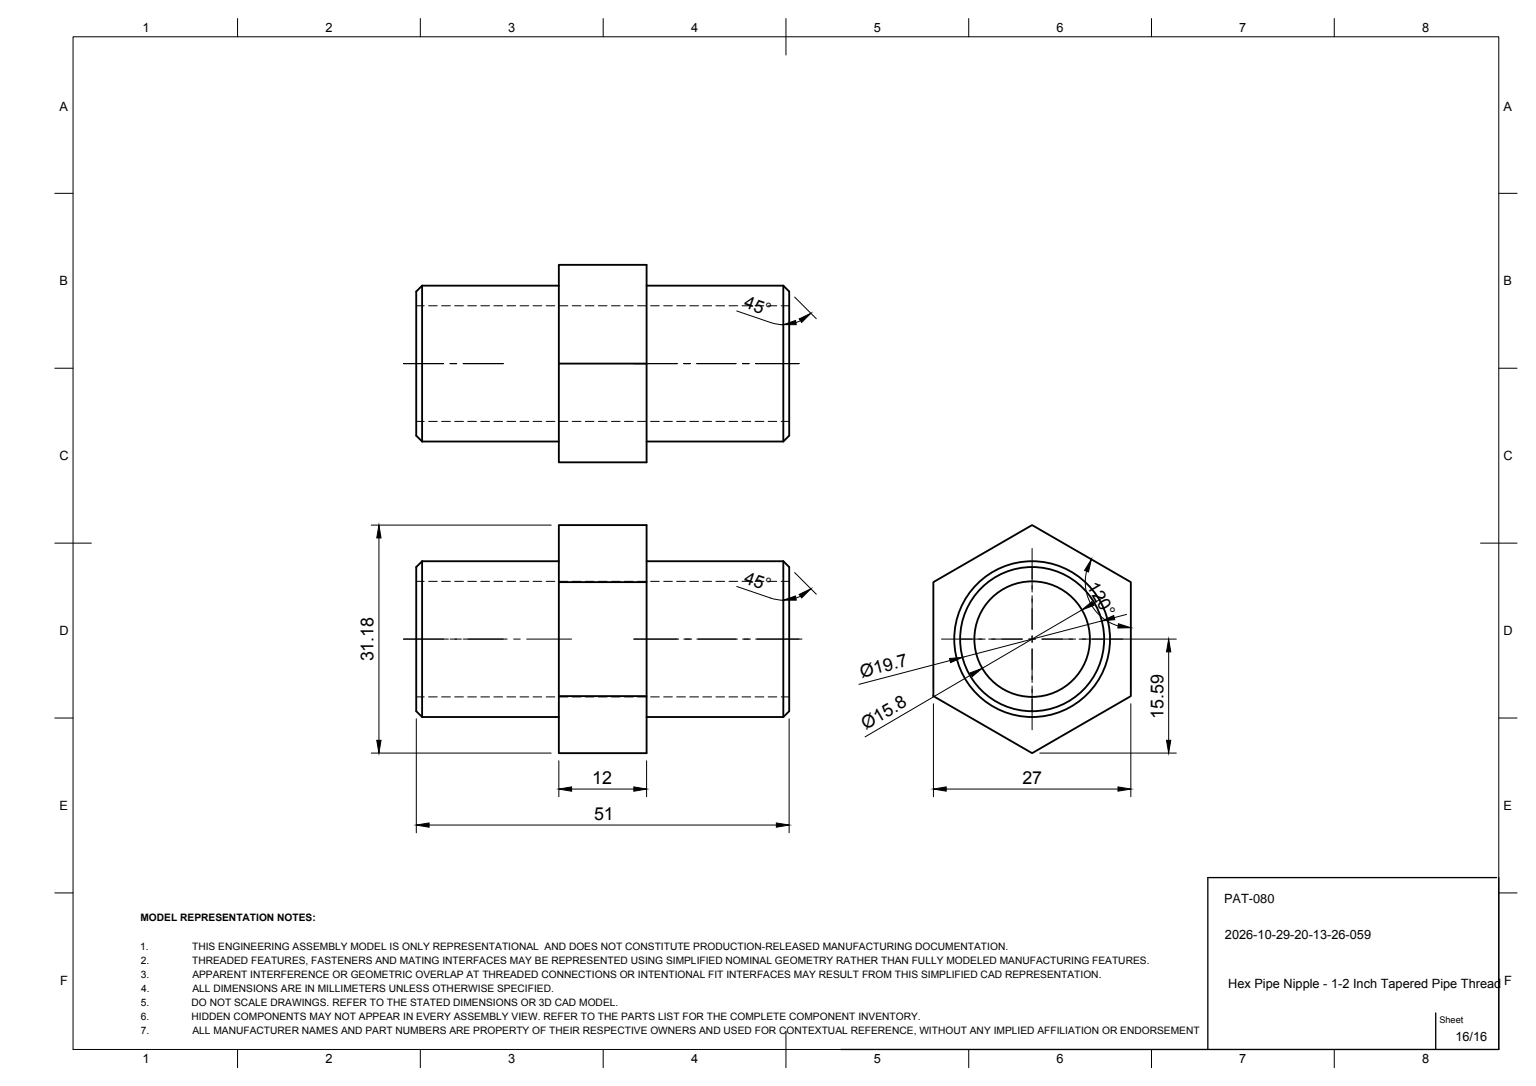
ISO-10303-21;
HEADER;
/* Generated by software containing ST-Developer
 * from STEP Tools, Inc. (www.steptools.com) 
 */

FILE_DESCRIPTION(
/* description */ ('PAT-080'),
/* implementation_level */ '2;1');

FILE_NAME(
/* name */ 'Hex Pipe Nipple - 1-2 Inch Tapered Pipe Thread.step',
/* time_stamp */ '2026-10-29T20:13:47-07:00',
/* author */ (''),
/* organization */ (''),
/* preprocessor_version */ 'ST-DEVELOPER v20.2',
/* originating_system */ 'Autodesk Translation Framework v15.17.0.0',
/* authorisation */ '');

FILE_SCHEMA (('AUTOMOTIVE_DESIGN { 1 0 10303 214 3 1 1 }'));
ENDSEC;

DATA;
#10=MECHANICAL_DESIGN_GEOMETRIC_PRESENTATION_REPRESENTATION('',(#261),#6878);
#194=CONICAL_SURFACE('',#4435,1.025,0.785398163397448);
#195=CONICAL_SURFACE('',#4438,1.025,0.785398163397448);
#223=SHAPE_REPRESENTATION_RELATIONSHIP('SRR','None',#6979,#242);
#242=ADVANCED_BREP_SHAPE_REPRESENTATION('',(#278),#6874);
#261=STYLED_ITEM('',(#7115),#278);
#278=MANIFOLD_SOLID_BREP('Body1',#3879);
#348=FACE_BOUND('',#973,.T.);
#349=FACE_BOUND('',#975,.T.);
#350=FACE_BOUND('',#984,.T.);
#351=FACE_BOUND('',#989,.T.);
#469=PLANE('',#4420);
#470=PLANE('',#4422);
#471=PLANE('',#4424);
#472=PLANE('',#4425);
#473=PLANE('',#4426);
#474=PLANE('',#4427);
#475=PLANE('',#4428);
#476=PLANE('',#4429);
#477=PLANE('',#4432);
#478=PLANE('',#4440);
#679=FACE_OUTER_BOUND('',#972,.T.);
#680=FACE_OUTER_BOUND('',#974,.T.);
#681=FACE_OUTER_BOUND('',#976,.T.);
#682=FACE_OUTER_BOUND('',#977,.T.);
#683=FACE_OUTER_BOUND('',#978,.T.);
#684=FACE_OUTER_BOUND('',#979,.T.);
#685=FACE_OUTER_BOUND('',#980,.T.);
#686=FACE_OUTER_BOUND('',#981,.T.);
#687=FACE_OUTER_BOUND('',#982,.T.);
#688=FACE_OUTER_BOUND('',#983,.T.);
#689=FACE_OUTER_BOUND('',#985,.T.);
#690=FACE_OUTER_BOUND('',#986,.T.);
#691=FACE_OUTER_BOUND('',#987,.T.);
#692=FACE_OUTER_BOUND('',#988,.T.);
#693=FACE_OUTER_BOUND('',#990,.T.);
#972=EDGE_LOOP('',(#3382,#3383,#3384,#3385,#3386,#3387));
#973=EDGE_LOOP('',(#3388));
#974=EDGE_LOOP('',(#3389,#3390,#3391,#3392,#3393,#3394));
#975=EDGE_LOOP('',(#3395));
#976=EDGE_LOOP('',(#3396,#3397,#3398,#3399));
#977=EDGE_LOOP('',(#3400,#3401,#3402,#3403));
#978=EDGE_LOOP('',(#3404,#3405,#3406,#3407));
#979=EDGE_LOOP('',(#3408,#3409,#3410,#3411));
#980=EDGE_LOOP('',(#3412,#3413,#3414,#3415));
#981=EDGE_LOOP('',(#3416,#3417,#3418,#3419));
#982=EDGE_LOOP('',(#3420,#3421,#3422,#3423));
#983=EDGE_LOOP('',(#3424));
#984=EDGE_LOOP('',(#3425));
#985=EDGE_LOOP('',(#3426,#3427,#3428,#3429));
#986=EDGE_LOOP('',(#3430,#3431,#3432,#3433));
#987=EDGE_LOOP('',(#3434,#3435,#3436,#3437));
#988=EDGE_LOOP('',(#3438));
#989=EDGE_LOOP('',(#3439));
#990=EDGE_LOOP('',(#3440,#3441,#3442,#3443));
#1285=LINE('',#6572,#1600);
#1286=LINE('',#6574,#1601);
#1287=LINE('',#6576,#1602);
#1288=LINE('',#6578,#1603);
#1289=LINE('',#6580,#1604);
#1290=LINE('',#6581,#1605);
#1291=LINE('',#6587,#1606);
#1292=LINE('',#6589,#1607);
#1293=LINE('',#6591,#1608);
#1294=LINE('',#6593,#1609);
#1295=LINE('',#6595,#1610);
#1296=LINE('',#6596,#1611);
#1297=LINE('',#6600,#1612);
#1298=LINE('',#6601,#1613);
#1299=LINE('',#6603,#1614);
#1300=LINE('',#6605,#1615);
#1301=LINE('',#6607,#1616);
#1302=LINE('',#6609,#1617);
#1303=LINE('',#6613,#1618);
#1304=LINE('',#6621,#1619);
#1305=LINE('',#6625,#1620);
#1306=LINE('',#6629,#1621);
#1307=LINE('',#6634,#1622);
#1600=VECTOR('',#5445,1.);
#1601=VECTOR('',#5446,1.);
#1602=VECTOR('',#5447,1.);
#1603=VECTOR('',#5448,1.);
#1604=VECTOR('',#5449,1.);
#1605=VECTOR('',#5450,1.);
#1606=VECTOR('',#5455,1.);
#1607=VECTOR('',#5456,1.);
#1608=VECTOR('',#5457,1.);
#1609=VECTOR('',#5458,1.);
#1610=VECTOR('',#5459,1.);
#1611=VECTOR('',#5460,1.);
#1612=VECTOR('',#5465,1.);
#1613=VECTOR('',#5466,1.);
#1614=VECTOR('',#5469,1.);
#1615=VECTOR('',#5472,1.);
#1616=VECTOR('',#5475,1.);
#1617=VECTOR('',#5478,1.);
#1618=VECTOR('',#5483,1.065);
#1619=VECTOR('',#5494,1.025);
#1620=VECTOR('',#5499,1.065);
#1621=VECTOR('',#5504,1.025);
#1622=VECTOR('',#5511,0.79);
#1786=CIRCLE('',#4421,1.065);
#1787=CIRCLE('',#4423,1.065);
#1788=CIRCLE('',#4431,1.065);
#1789=CIRCLE('',#4433,0.985);
#1790=CIRCLE('',#4434,0.79);
#1791=CIRCLE('',#4437,1.065);
#1792=CIRCLE('',#4439,0.985);
#1793=CIRCLE('',#4441,0.79);
#2067=VERTEX_POINT('',#6570);
#2068=VERTEX_POINT('',#6571);
#2069=VERTEX_POINT('',#6573);
#2070=VERTEX_POINT('',#6575);
#2071=VERTEX_POINT('',#6577);
#2072=VERTEX_POINT('',#6579);
#2073=VERTEX_POINT('',#6582);
#2074=VERTEX_POINT('',#6585);
#2075=VERTEX_POINT('',#6586);
#2076=VERTEX_POINT('',#6588);
#2077=VERTEX_POINT('',#6590);
#2078=VERTEX_POINT('',#6592);
#2079=VERTEX_POINT('',#6594);
#2080=VERTEX_POINT('',#6597);
#2081=VERTEX_POINT('',#6612);
#2082=VERTEX_POINT('',#6616);
#2083=VERTEX_POINT('',#6618);
#2084=VERTEX_POINT('',#6623);
#2085=VERTEX_POINT('',#6627);
#2086=VERTEX_POINT('',#6631);
#2514=EDGE_CURVE('',#2067,#2068,#1285,.T.);
#2515=EDGE_CURVE('',#2068,#2069,#1286,.T.);
#2516=EDGE_CURVE('',#2069,#2070,#1287,.T.);
#2517=EDGE_CURVE('',#2070,#2071,#1288,.T.);
#2518=EDGE_CURVE('',#2071,#2072,#1289,.T.);
#2519=EDGE_CURVE('',#2072,#2067,#1290,.T.);
#2520=EDGE_CURVE('',#2073,#2073,#1786,.T.);
#2521=EDGE_CURVE('',#2074,#2075,#1291,.T.);
#2522=EDGE_CURVE('',#2075,#2076,#1292,.T.);
#2523=EDGE_CURVE('',#2076,#2077,#1293,.T.);
#2524=EDGE_CURVE('',#2077,#2078,#1294,.T.);
#2525=EDGE_CURVE('',#2078,#2079,#1295,.T.);
#2526=EDGE_CURVE('',#2079,#2074,#1296,.T.);
#2527=EDGE_CURVE('',#2080,#2080,#1787,.T.);
#2528=EDGE_CURVE('',#2074,#2068,#1297,.T.);
#2529=EDGE_CURVE('',#2069,#2079,#1298,.T.);
#2530=EDGE_CURVE('',#2070,#2078,#1299,.T.);
#2531=EDGE_CURVE('',#2071,#2077,#1300,.T.);
#2532=EDGE_CURVE('',#2072,#2076,#1301,.T.);
#2533=EDGE_CURVE('',#2067,#2075,#1302,.T.);
#2534=EDGE_CURVE('',#2080,#2081,#1303,.T.);
#2535=EDGE_CURVE('',#2081,#2081,#1788,.T.);
#2536=EDGE_CURVE('',#2082,#2082,#1789,.T.);
#2537=EDGE_CURVE('',#2083,#2083,#1790,.T.);
#2538=EDGE_CURVE('',#2081,#2082,#1304,.T.);
#2539=EDGE_CURVE('',#2084,#2084,#1791,.T.);
#2540=EDGE_CURVE('',#2084,#2073,#1305,.T.);
#2541=EDGE_CURVE('',#2085,#2085,#1792,.T.);
#2542=EDGE_CURVE('',#2085,#2084,#1306,.T.);
#2543=EDGE_CURVE('',#2086,#2086,#1793,.T.);
#2544=EDGE_CURVE('',#2086,#2083,#1307,.T.);
#3382=ORIENTED_EDGE('',*,*,#2514,.T.);
#3383=ORIENTED_EDGE('',*,*,#2515,.T.);
#3384=ORIENTED_EDGE('',*,*,#2516,.T.);
#3385=ORIENTED_EDGE('',*,*,#2517,.T.);
#3386=ORIENTED_EDGE('',*,*,#2518,.T.);
#3387=ORIENTED_EDGE('',*,*,#2519,.T.);
#3388=ORIENTED_EDGE('',*,*,#2520,.F.);
#3389=ORIENTED_EDGE('',*,*,#2521,.T.);
#3390=ORIENTED_EDGE('',*,*,#2522,.T.);
#3391=ORIENTED_EDGE('',*,*,#2523,.T.);
#3392=ORIENTED_EDGE('',*,*,#2524,.T.);
#3393=ORIENTED_EDGE('',*,*,#2525,.T.);
#3394=ORIENTED_EDGE('',*,*,#2526,.T.);
#3395=ORIENTED_EDGE('',*,*,#2527,.F.);
#3396=ORIENTED_EDGE('',*,*,#2528,.F.);
#3397=ORIENTED_EDGE('',*,*,#2526,.F.);
#3398=ORIENTED_EDGE('',*,*,#2529,.F.);
#3399=ORIENTED_EDGE('',*,*,#2515,.F.);
#3400=ORIENTED_EDGE('',*,*,#2529,.T.);
#3401=ORIENTED_EDGE('',*,*,#2525,.F.);
#3402=ORIENTED_EDGE('',*,*,#2530,.F.);
#3403=ORIENTED_EDGE('',*,*,#2516,.F.);
#3404=ORIENTED_EDGE('',*,*,#2530,.T.);
#3405=ORIENTED_EDGE('',*,*,#2524,.F.);
#3406=ORIENTED_EDGE('',*,*,#2531,.F.);
#3407=ORIENTED_EDGE('',*,*,#2517,.F.);
#3408=ORIENTED_EDGE('',*,*,#2531,.T.);
#3409=ORIENTED_EDGE('',*,*,#2523,.F.);
#3410=ORIENTED_EDGE('',*,*,#2532,.F.);
#3411=ORIENTED_EDGE('',*,*,#2518,.F.);
#3412=ORIENTED_EDGE('',*,*,#2532,.T.);
#3413=ORIENTED_EDGE('',*,*,#2522,.F.);
#3414=ORIENTED_EDGE('',*,*,#2533,.F.);
#3415=ORIENTED_EDGE('',*,*,#2519,.F.);
#3416=ORIENTED_EDGE('',*,*,#2533,.T.);
#3417=ORIENTED_EDGE('',*,*,#2521,.F.);
#3418=ORIENTED_EDGE('',*,*,#2528,.T.);
#3419=ORIENTED_EDGE('',*,*,#2514,.F.);
#3420=ORIENTED_EDGE('',*,*,#2527,.T.);
#3421=ORIENTED_EDGE('',*,*,#2534,.T.);
#3422=ORIENTED_EDGE('',*,*,#2535,.T.);
#3423=ORIENTED_EDGE('',*,*,#2534,.F.);
#3424=ORIENTED_EDGE('',*,*,#2536,.F.);
#3425=ORIENTED_EDGE('',*,*,#2537,.T.);
#3426=ORIENTED_EDGE('',*,*,#2535,.F.);
#3427=ORIENTED_EDGE('',*,*,#2538,.T.);
#3428=ORIENTED_EDGE('',*,*,#2536,.T.);
#3429=ORIENTED_EDGE('',*,*,#2538,.F.);
#3430=ORIENTED_EDGE('',*,*,#2539,.F.);
#3431=ORIENTED_EDGE('',*,*,#2540,.T.);
#3432=ORIENTED_EDGE('',*,*,#2520,.T.);
#3433=ORIENTED_EDGE('',*,*,#2540,.F.);
#3434=ORIENTED_EDGE('',*,*,#2541,.F.);
#3435=ORIENTED_EDGE('',*,*,#2542,.T.);
#3436=ORIENTED_EDGE('',*,*,#2539,.T.);
#3437=ORIENTED_EDGE('',*,*,#2542,.F.);
#3438=ORIENTED_EDGE('',*,*,#2541,.T.);
#3439=ORIENTED_EDGE('',*,*,#2543,.F.);
#3440=ORIENTED_EDGE('',*,*,#2543,.T.);
#3441=ORIENTED_EDGE('',*,*,#2544,.T.);
#3442=ORIENTED_EDGE('',*,*,#2537,.F.);
#3443=ORIENTED_EDGE('',*,*,#2544,.F.);
#3628=CYLINDRICAL_SURFACE('',#4430,1.065);
#3629=CYLINDRICAL_SURFACE('',#4436,1.065);
#3630=CYLINDRICAL_SURFACE('',#4442,0.79);
#3815=ADVANCED_FACE('',(#679,#348),#469,.F.);
#3816=ADVANCED_FACE('',(#680,#349),#470,.T.);
#3817=ADVANCED_FACE('',(#681),#471,.T.);
#3818=ADVANCED_FACE('',(#682),#472,.T.);
#3819=ADVANCED_FACE('',(#683),#473,.T.);
#3820=ADVANCED_FACE('',(#684),#474,.T.);
#3821=ADVANCED_FACE('',(#685),#475,.T.);
#3822=ADVANCED_FACE('',(#686),#476,.T.);
#3823=ADVANCED_FACE('',(#687),#3628,.T.);
#3824=ADVANCED_FACE('',(#688,#350),#477,.T.);
#3825=ADVANCED_FACE('',(#689),#194,.T.);
#3826=ADVANCED_FACE('',(#690),#3629,.T.);
#3827=ADVANCED_FACE('',(#691),#195,.T.);
#3828=ADVANCED_FACE('',(#692,#351),#478,.T.);
#3829=ADVANCED_FACE('',(#693),#3630,.F.);
#3879=CLOSED_SHELL('',(#3815,#3816,#3817,#3818,#3819,#3820,#3821,#3822,
#3823,#3824,#3825,#3826,#3827,#3828,#3829));
#4419=AXIS2_PLACEMENT_3D('',#6568,#5441,#5442);
#4420=AXIS2_PLACEMENT_3D('',#6569,#5443,#5444);
#4421=AXIS2_PLACEMENT_3D('',#6583,#5451,#5452);
#4422=AXIS2_PLACEMENT_3D('',#6584,#5453,#5454);
#4423=AXIS2_PLACEMENT_3D('',#6598,#5461,#5462);
#4424=AXIS2_PLACEMENT_3D('',#6599,#5463,#5464);
#4425=AXIS2_PLACEMENT_3D('',#6602,#5467,#5468);
#4426=AXIS2_PLACEMENT_3D('',#6604,#5470,#5471);
#4427=AXIS2_PLACEMENT_3D('',#6606,#5473,#5474);
#4428=AXIS2_PLACEMENT_3D('',#6608,#5476,#5477);
#4429=AXIS2_PLACEMENT_3D('',#6610,#5479,#5480);
#4430=AXIS2_PLACEMENT_3D('',#6611,#5481,#5482);
#4431=AXIS2_PLACEMENT_3D('',#6614,#5484,#5485);
#4432=AXIS2_PLACEMENT_3D('',#6615,#5486,#5487);
#4433=AXIS2_PLACEMENT_3D('',#6617,#5488,#5489);
#4434=AXIS2_PLACEMENT_3D('',#6619,#5490,#5491);
#4435=AXIS2_PLACEMENT_3D('',#6620,#5492,#5493);
#4436=AXIS2_PLACEMENT_3D('',#6622,#5495,#5496);
#4437=AXIS2_PLACEMENT_3D('',#6624,#5497,#5498);
#4438=AXIS2_PLACEMENT_3D('',#6626,#5500,#5501);
#4439=AXIS2_PLACEMENT_3D('',#6628,#5502,#5503);
#4440=AXIS2_PLACEMENT_3D('',#6630,#5505,#5506);
#4441=AXIS2_PLACEMENT_3D('',#6632,#5507,#5508);
#4442=AXIS2_PLACEMENT_3D('',#6633,#5509,#5510);
#5441=DIRECTION('axis',(0.,0.,1.));
#5442=DIRECTION('refdir',(1.,0.,0.));
#5443=DIRECTION('center_axis',(0.,1.,0.));
#5444=DIRECTION('ref_axis',(1.,0.,0.));
#5445=DIRECTION('',(-0.5,0.,0.866025403784439));
#5446=DIRECTION('',(-1.,0.,-2.84883360945713E-16));
#5447=DIRECTION('',(-0.5,0.,-0.866025403784439));
#5448=DIRECTION('',(0.5,0.,-0.866025403784439));
#5449=DIRECTION('',(1.,0.,0.));
#5450=DIRECTION('',(0.5,0.,0.866025403784439));
#5451=DIRECTION('center_axis',(0.,-1.,0.));
#5452=DIRECTION('ref_axis',(1.,0.,0.));
#5453=DIRECTION('center_axis',(0.,1.,0.));
#5454=DIRECTION('ref_axis',(1.,0.,0.));
#5455=DIRECTION('',(0.5,0.,-0.866025403784439));
#5456=DIRECTION('',(-0.5,0.,-0.866025403784439));
#5457=DIRECTION('',(-1.,0.,0.));
#5458=DIRECTION('',(-0.5,0.,0.866025403784439));
#5459=DIRECTION('',(0.5,0.,0.866025403784439));
#5460=DIRECTION('',(1.,0.,2.84883360945713E-16));
#5461=DIRECTION('center_axis',(0.,1.,0.));
#5462=DIRECTION('ref_axis',(1.,0.,0.));
#5463=DIRECTION('center_axis',(-2.84883360945713E-16,0.,1.));
#5464=DIRECTION('ref_axis',(1.,0.,2.84883360945713E-16));
#5465=DIRECTION('',(0.,-1.,0.));
#5466=DIRECTION('',(0.,1.,0.));
#5467=DIRECTION('center_axis',(-0.866025403784439,0.,0.5));
#5468=DIRECTION('ref_axis',(0.5,0.,0.866025403784439));
#5469=DIRECTION('',(0.,1.,0.));
#5470=DIRECTION('center_axis',(-0.866025403784439,0.,-0.5));
#5471=DIRECTION('ref_axis',(-0.5,0.,0.866025403784439));
#5472=DIRECTION('',(0.,1.,0.));
#5473=DIRECTION('center_axis',(0.,0.,-1.));
#5474=DIRECTION('ref_axis',(-1.,0.,0.));
#5475=DIRECTION('',(0.,1.,0.));
#5476=DIRECTION('center_axis',(0.866025403784439,0.,-0.5));
#5477=DIRECTION('ref_axis',(-0.5,0.,-0.866025403784439));
#5478=DIRECTION('',(0.,1.,0.));
#5479=DIRECTION('center_axis',(0.866025403784439,0.,0.5));
#5480=DIRECTION('ref_axis',(0.5,0.,-0.866025403784439));
#5481=DIRECTION('center_axis',(0.,-1.,0.));
#5482=DIRECTION('ref_axis',(1.,0.,0.));
#5483=DIRECTION('',(0.,1.,0.));
#5484=DIRECTION('center_axis',(0.,-1.,0.));
#5485=DIRECTION('ref_axis',(1.,0.,0.));
#5486=DIRECTION('center_axis',(0.,1.,0.));
#5487=DIRECTION('ref_axis',(0.,0.,1.));
#5488=DIRECTION('center_axis',(0.,-1.,0.));
#5489=DIRECTION('ref_axis',(1.,0.,0.));
#5490=DIRECTION('center_axis',(0.,-1.,0.));
#5491=DIRECTION('ref_axis',(1.,0.,0.));
#5492=DIRECTION('center_axis',(0.,-1.,0.));
#5493=DIRECTION('ref_axis',(1.,0.,0.));
#5494=DIRECTION('',(0.707106781186547,0.707106781186548,8.65956056235493E-17));
#5495=DIRECTION('center_axis',(0.,-1.,0.));
#5496=DIRECTION('ref_axis',(1.,0.,0.));
#5497=DIRECTION('center_axis',(0.,-1.,0.));
#5498=DIRECTION('ref_axis',(1.,0.,0.));
#5499=DIRECTION('',(0.,1.,0.));
#5500=DIRECTION('center_axis',(0.,1.,0.));
#5501=DIRECTION('ref_axis',(1.,0.,0.));
#5502=DIRECTION('center_axis',(0.,-1.,0.));
#5503=DIRECTION('ref_axis',(1.,0.,0.));
#5504=DIRECTION('',(-0.707106781186547,0.707106781186548,-8.65956056235493E-17));
#5505=DIRECTION('center_axis',(0.,-1.,0.));
#5506=DIRECTION('ref_axis',(0.,0.,-1.));
#5507=DIRECTION('center_axis',(0.,-1.,0.));
#5508=DIRECTION('ref_axis',(1.,0.,0.));
#5509=DIRECTION('center_axis',(0.,-1.,0.));
#5510=DIRECTION('ref_axis',(1.,0.,0.));
#5511=DIRECTION('',(0.,1.,0.));
#6568=CARTESIAN_POINT('',(0.,0.,0.));
#6569=CARTESIAN_POINT('Origin',(0.,-0.6,0.));
#6570=CARTESIAN_POINT('',(1.55884572681199,-0.6,0.));
#6571=CARTESIAN_POINT('',(0.779422863405995,-0.6,1.35));
#6572=CARTESIAN_POINT('',(0.779422863405995,-0.6,1.35));
#6573=CARTESIAN_POINT('',(-0.779422863405996,-0.6,1.35));
#6574=CARTESIAN_POINT('',(-0.779422863405996,-0.6,1.35));
#6575=CARTESIAN_POINT('',(-1.55884572681199,-0.6,-1.90903542970483E-16));
#6576=CARTESIAN_POINT('',(-1.55884572681199,-0.6,-1.90903542970483E-16));
#6577=CARTESIAN_POINT('',(-0.779422863405995,-0.6,-1.35));
#6578=CARTESIAN_POINT('',(-0.779422863405995,-0.6,-1.35));
#6579=CARTESIAN_POINT('',(0.779422863405995,-0.6,-1.35));
#6580=CARTESIAN_POINT('',(0.779422863405995,-0.6,-1.35));
#6581=CARTESIAN_POINT('',(1.55884572681199,-0.6,0.));
#6582=CARTESIAN_POINT('',(-1.065,-0.6,-1.30424884109193E-16));
#6583=CARTESIAN_POINT('Origin',(0.,-0.6,0.));
#6584=CARTESIAN_POINT('Origin',(0.,0.6,0.));
#6585=CARTESIAN_POINT('',(0.779422863405995,0.6,1.35));
#6586=CARTESIAN_POINT('',(1.55884572681199,0.6,0.));
#6587=CARTESIAN_POINT('',(0.779422863405995,0.6,1.35));
#6588=CARTESIAN_POINT('',(0.779422863405995,0.6,-1.35));
#6589=CARTESIAN_POINT('',(1.55884572681199,0.6,0.));
#6590=CARTESIAN_POINT('',(-0.779422863405995,0.6,-1.35));
#6591=CARTESIAN_POINT('',(0.779422863405995,0.6,-1.35));
#6592=CARTESIAN_POINT('',(-1.55884572681199,0.6,-1.90903542970483E-16));
#6593=CARTESIAN_POINT('',(-0.779422863405995,0.6,-1.35));
#6594=CARTESIAN_POINT('',(-0.779422863405996,0.6,1.35));
#6595=CARTESIAN_POINT('',(-1.55884572681199,0.6,-1.90903542970483E-16));
#6596=CARTESIAN_POINT('',(-0.779422863405996,0.6,1.35));
#6597=CARTESIAN_POINT('',(-1.065,0.6,1.30424884109193E-16));
#6598=CARTESIAN_POINT('Origin',(0.,0.6,0.));
#6599=CARTESIAN_POINT('Origin',(-0.779422863405996,0.,1.35));
#6600=CARTESIAN_POINT('',(0.779422863405995,0.,1.35));
#6601=CARTESIAN_POINT('',(-0.779422863405996,0.,1.35));
#6602=CARTESIAN_POINT('Origin',(-1.55884572681199,0.,-1.90903542970483E-16));
#6603=CARTESIAN_POINT('',(-1.55884572681199,0.,-1.90903542970483E-16));
#6604=CARTESIAN_POINT('Origin',(-0.779422863405995,0.,-1.35));
#6605=CARTESIAN_POINT('',(-0.779422863405995,0.,-1.35));
#6606=CARTESIAN_POINT('Origin',(0.779422863405995,0.,-1.35));
#6607=CARTESIAN_POINT('',(0.779422863405995,0.,-1.35));
#6608=CARTESIAN_POINT('Origin',(1.55884572681199,0.,0.));
#6609=CARTESIAN_POINT('',(1.55884572681199,0.,0.));
#6610=CARTESIAN_POINT('Origin',(0.779422863405995,0.,1.35));
#6611=CARTESIAN_POINT('Origin',(0.,0.,0.));
#6612=CARTESIAN_POINT('',(-1.065,2.47,-1.30424884109193E-16));
#6613=CARTESIAN_POINT('',(-1.065,0.,-1.30424884109193E-16));
#6614=CARTESIAN_POINT('Origin',(0.,2.47,0.));
#6615=CARTESIAN_POINT('Origin',(0.985,2.55,0.));
#6616=CARTESIAN_POINT('',(-0.985,2.55,-1.20627709716014E-16));
#6617=CARTESIAN_POINT('Origin',(0.,2.55,0.));
#6618=CARTESIAN_POINT('',(-0.79,2.55,-9.67470971326409E-17));
#6619=CARTESIAN_POINT('Origin',(0.,2.55,0.));
#6620=CARTESIAN_POINT('Origin',(0.,2.51,0.));
#6621=CARTESIAN_POINT('',(-1.025,2.51,-1.25526296912604E-16));
#6622=CARTESIAN_POINT('Origin',(0.,0.,0.));
#6623=CARTESIAN_POINT('',(-1.065,-2.47,-1.30424884109193E-16));
#6624=CARTESIAN_POINT('Origin',(0.,-2.47,0.));
#6625=CARTESIAN_POINT('',(-1.065,0.,-1.30424884109193E-16));
#6626=CARTESIAN_POINT('Origin',(0.,-2.51,0.));
#6627=CARTESIAN_POINT('',(-0.985,-2.55,-1.20627709716014E-16));
#6628=CARTESIAN_POINT('Origin',(0.,-2.55,0.));
#6629=CARTESIAN_POINT('',(-1.025,-2.51,-1.25526296912604E-16));
#6630=CARTESIAN_POINT('Origin',(0.79,-2.55,0.));
#6631=CARTESIAN_POINT('',(-0.79,-2.55,-9.67470971326409E-17));
#6632=CARTESIAN_POINT('Origin',(0.,-2.55,0.));
#6633=CARTESIAN_POINT('Origin',(0.,0.,0.));
#6634=CARTESIAN_POINT('',(-0.79,0.,-9.67470971326409E-17));
#6853=UNCERTAINTY_MEASURE_WITH_UNIT(LENGTH_MEASURE(0.001),#6879,
'DISTANCE_ACCURACY_VALUE',
'Maximum model space distance between geometric entities at asserted c
onnectivities');
#6857=UNCERTAINTY_MEASURE_WITH_UNIT(LENGTH_MEASURE(0.001),#6879,
'DISTANCE_ACCURACY_VALUE',
'Maximum model space distance between geometric entities at asserted c
onnectivities');
#6874=(
GEOMETRIC_REPRESENTATION_CONTEXT(3)
GLOBAL_UNCERTAINTY_ASSIGNED_CONTEXT((#6853))
GLOBAL_UNIT_ASSIGNED_CONTEXT((#6879,#6881,#6882))
REPRESENTATION_CONTEXT('','3D')
);
#6878=(
GEOMETRIC_REPRESENTATION_CONTEXT(3)
GLOBAL_UNCERTAINTY_ASSIGNED_CONTEXT((#6857))
GLOBAL_UNIT_ASSIGNED_CONTEXT((#6879,#6881,#6882))
REPRESENTATION_CONTEXT('','3D')
);
#6879=(
LENGTH_UNIT()
NAMED_UNIT(*)
SI_UNIT(.CENTI.,.METRE.)
);
#6881=(
NAMED_UNIT(*)
PLANE_ANGLE_UNIT()
SI_UNIT($,.RADIAN.)
);
#6882=(
NAMED_UNIT(*)
SI_UNIT($,.STERADIAN.)
SOLID_ANGLE_UNIT()
);
#6899=SHAPE_DEFINITION_REPRESENTATION(#6919,#6979);
#6919=PRODUCT_DEFINITION_SHAPE('',$,#7000);
#6979=SHAPE_REPRESENTATION('',(#4419),#6874);
#6983=PRODUCT_DEFINITION_CONTEXT('part definition',#7045,'design');
#7000=PRODUCT_DEFINITION('Hex Pipe Nipple - 1-2 Inch Tapered Pipe Thread',
'Hex Pipe Nipple - 1-2 Inch Tapered Pipe Thread',#7020,#6983);
#7020=PRODUCT_DEFINITION_FORMATION('',$,#7063);
#7045=APPLICATION_CONTEXT(
'Core Data for Automotive Mechanical Design Process');
#7046=PRODUCT_CONTEXT('part definition',#7045,'mechanical');
#7063=PRODUCT('Hex Pipe Nipple - 1-2 Inch Tapered Pipe Thread',
'Hex Pipe Nipple - 1-2 Inch Tapered Pipe Thread',
'Hex Pipe Nipple - 1-2 Inch Tapered Pipe Thread',(#7046));
#7109=COLOUR_RGB('Light Blue',0.38,0.62,0.78);
#7110=FILL_AREA_STYLE_COLOUR('',#7109);
#7111=FILL_AREA_STYLE('',(#7110));
#7112=SURFACE_STYLE_FILL_AREA(#7111);
#7113=SURFACE_SIDE_STYLE('',(#7112));
#7114=SURFACE_STYLE_USAGE(.BOTH.,#7113);
#7115=PRESENTATION_STYLE_ASSIGNMENT((#7114));
ENDSEC;
END-ISO-10303-21;
